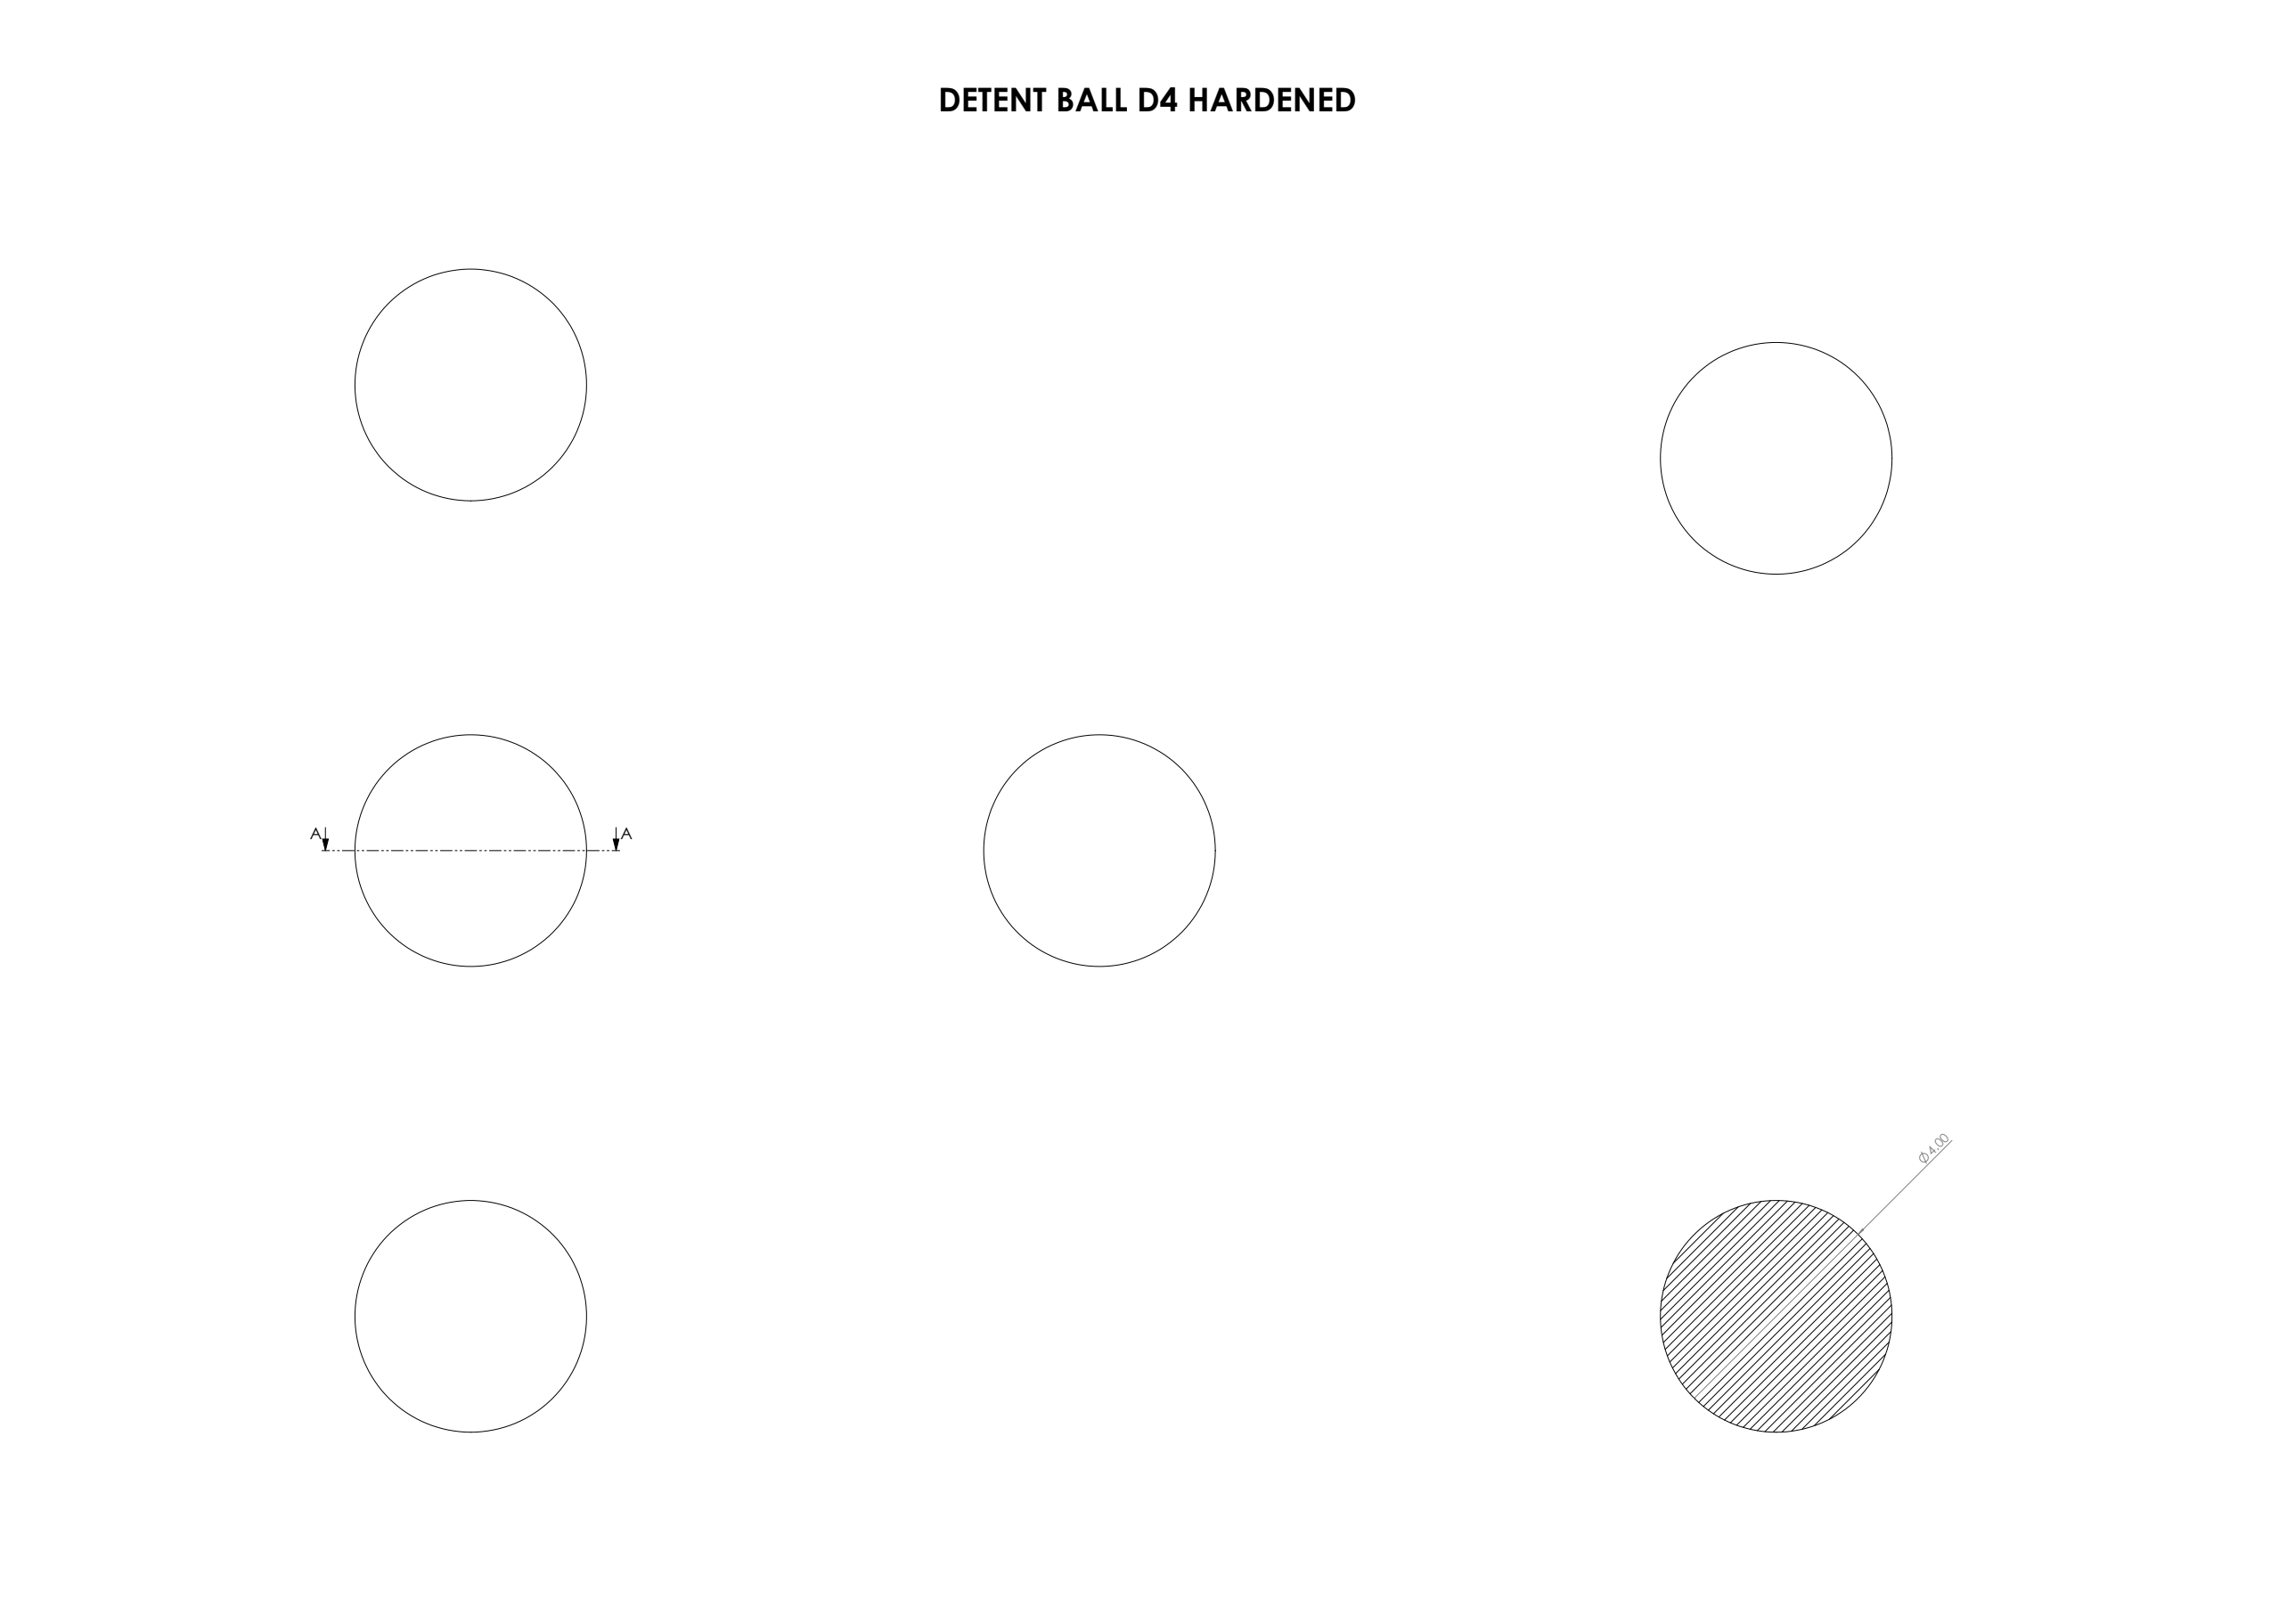
ISO-10303-21;
HEADER;
/* Generated by software containing ST-Developer
 * from STEP Tools, Inc. (www.steptools.com) 
 */

FILE_DESCRIPTION(
/* description */ (''),
/* implementation_level */ '2;1');

FILE_NAME(
/* name */ '09_Detent_Ball_D4_Hardened.step',
/* time_stamp */ '2026-10-21T02:03:06-07:00',
/* author */ (''),
/* organization */ (''),
/* preprocessor_version */ 'ST-DEVELOPER v20.2',
/* originating_system */ 'Autodesk Translation Framework v15.15.0.0',
/* authorisation */ '');

FILE_SCHEMA (('AUTOMOTIVE_DESIGN { 1 0 10303 214 3 1 1 }'));
ENDSEC;

DATA;
#10=MECHANICAL_DESIGN_GEOMETRIC_PRESENTATION_REPRESENTATION('',(#123),#38528);
#75=SPHERICAL_SURFACE('',#18767,2.);
#99=SHAPE_REPRESENTATION_RELATIONSHIP('SRR','None',#38584,#111);
#111=ADVANCED_BREP_SHAPE_REPRESENTATION('',(#135),#38524);
#123=STYLED_ITEM('',(#38720),#135);
#135=MANIFOLD_SOLID_BREP('Body1',#17080);
#2196=CIRCLE('',#18768,2.);
#3103=FACE_OUTER_BOUND('',#4129,.T.);
#4129=EDGE_LOOP('',(#14723,#14724));
#7585=VERTEX_POINT('',#33823);
#7586=VERTEX_POINT('',#33824);
#10013=EDGE_CURVE('',#7585,#7586,#2196,.T.);
#14723=ORIENTED_EDGE('',*,*,#10013,.T.);
#14724=ORIENTED_EDGE('',*,*,#10013,.F.);
#16912=ADVANCED_FACE('',(#3103),#75,.T.);
#17080=CLOSED_SHELL('',(#16912));
#18766=AXIS2_PLACEMENT_3D('',#33821,#22887,#22888);
#18767=AXIS2_PLACEMENT_3D('',#33822,#22889,#22890);
#18768=AXIS2_PLACEMENT_3D('',#33825,#22891,#22892);
#22887=DIRECTION('axis',(0.,0.,1.));
#22888=DIRECTION('refdir',(1.,0.,0.));
#22889=DIRECTION('center_axis',(6.12323399573677E-17,0.,1.));
#22890=DIRECTION('ref_axis',(1.,0.,0.));
#22891=DIRECTION('center_axis',(1.22464679914735E-16,-1.,0.));
#22892=DIRECTION('ref_axis',(-1.,-1.22464679914735E-16,0.));
#33821=CARTESIAN_POINT('',(0.,0.,0.));
#33822=CARTESIAN_POINT('Origin',(0.,0.,0.));
#33823=CARTESIAN_POINT('',(-1.22464679914735E-16,-1.49975978266186E-32,
2.));
#33824=CARTESIAN_POINT('',(-1.22464679914735E-16,-1.49975978266186E-32,
-2.));
#33825=CARTESIAN_POINT('Origin',(0.,0.,0.));
#38510=UNCERTAINTY_MEASURE_WITH_UNIT(LENGTH_MEASURE(0.01),#38529,
'DISTANCE_ACCURACY_VALUE',
'Maximum model space distance between geometric entities at asserted c
onnectivities');
#38514=UNCERTAINTY_MEASURE_WITH_UNIT(LENGTH_MEASURE(0.01),#38529,
'DISTANCE_ACCURACY_VALUE',
'Maximum model space distance between geometric entities at asserted c
onnectivities');
#38524=(
GEOMETRIC_REPRESENTATION_CONTEXT(3)
GLOBAL_UNCERTAINTY_ASSIGNED_CONTEXT((#38510))
GLOBAL_UNIT_ASSIGNED_CONTEXT((#38529,#38531,#38532))
REPRESENTATION_CONTEXT('','3D')
);
#38528=(
GEOMETRIC_REPRESENTATION_CONTEXT(3)
GLOBAL_UNCERTAINTY_ASSIGNED_CONTEXT((#38514))
GLOBAL_UNIT_ASSIGNED_CONTEXT((#38529,#38531,#38532))
REPRESENTATION_CONTEXT('','3D')
);
#38529=(
LENGTH_UNIT()
NAMED_UNIT(*)
SI_UNIT(.MILLI.,.METRE.)
);
#38531=(
NAMED_UNIT(*)
PLANE_ANGLE_UNIT()
SI_UNIT($,.RADIAN.)
);
#38532=(
NAMED_UNIT(*)
SI_UNIT($,.STERADIAN.)
SOLID_ANGLE_UNIT()
);
#38542=SHAPE_DEFINITION_REPRESENTATION(#38555,#38584);
#38555=PRODUCT_DEFINITION_SHAPE('',$,#38598);
#38584=SHAPE_REPRESENTATION('',(#18766),#38524);
#38588=PRODUCT_DEFINITION_CONTEXT('part definition',#38629,'design');
#38598=PRODUCT_DEFINITION('2026-10-20-13-39-10-336',
'09_Detent_Ball_D4_Hardened',#38611,#38588);
#38611=PRODUCT_DEFINITION_FORMATION('',$,#38640);
#38629=APPLICATION_CONTEXT(
'Core Data for Automotive Mechanical Design Process');
#38630=PRODUCT_CONTEXT('part definition',#38629,'mechanical');
#38640=PRODUCT('2026-10-20-13-39-10-336','09_Detent_Ball_D4_Hardened',$,
(#38630));
#38714=COLOUR_RGB('Off White',0.89,0.88,0.83);
#38715=FILL_AREA_STYLE_COLOUR('',#38714);
#38716=FILL_AREA_STYLE('',(#38715));
#38717=SURFACE_STYLE_FILL_AREA(#38716);
#38718=SURFACE_SIDE_STYLE('',(#38717));
#38719=SURFACE_STYLE_USAGE(.BOTH.,#38718);
#38720=PRESENTATION_STYLE_ASSIGNMENT((#38719));
ENDSEC;
END-ISO-10303-21;
